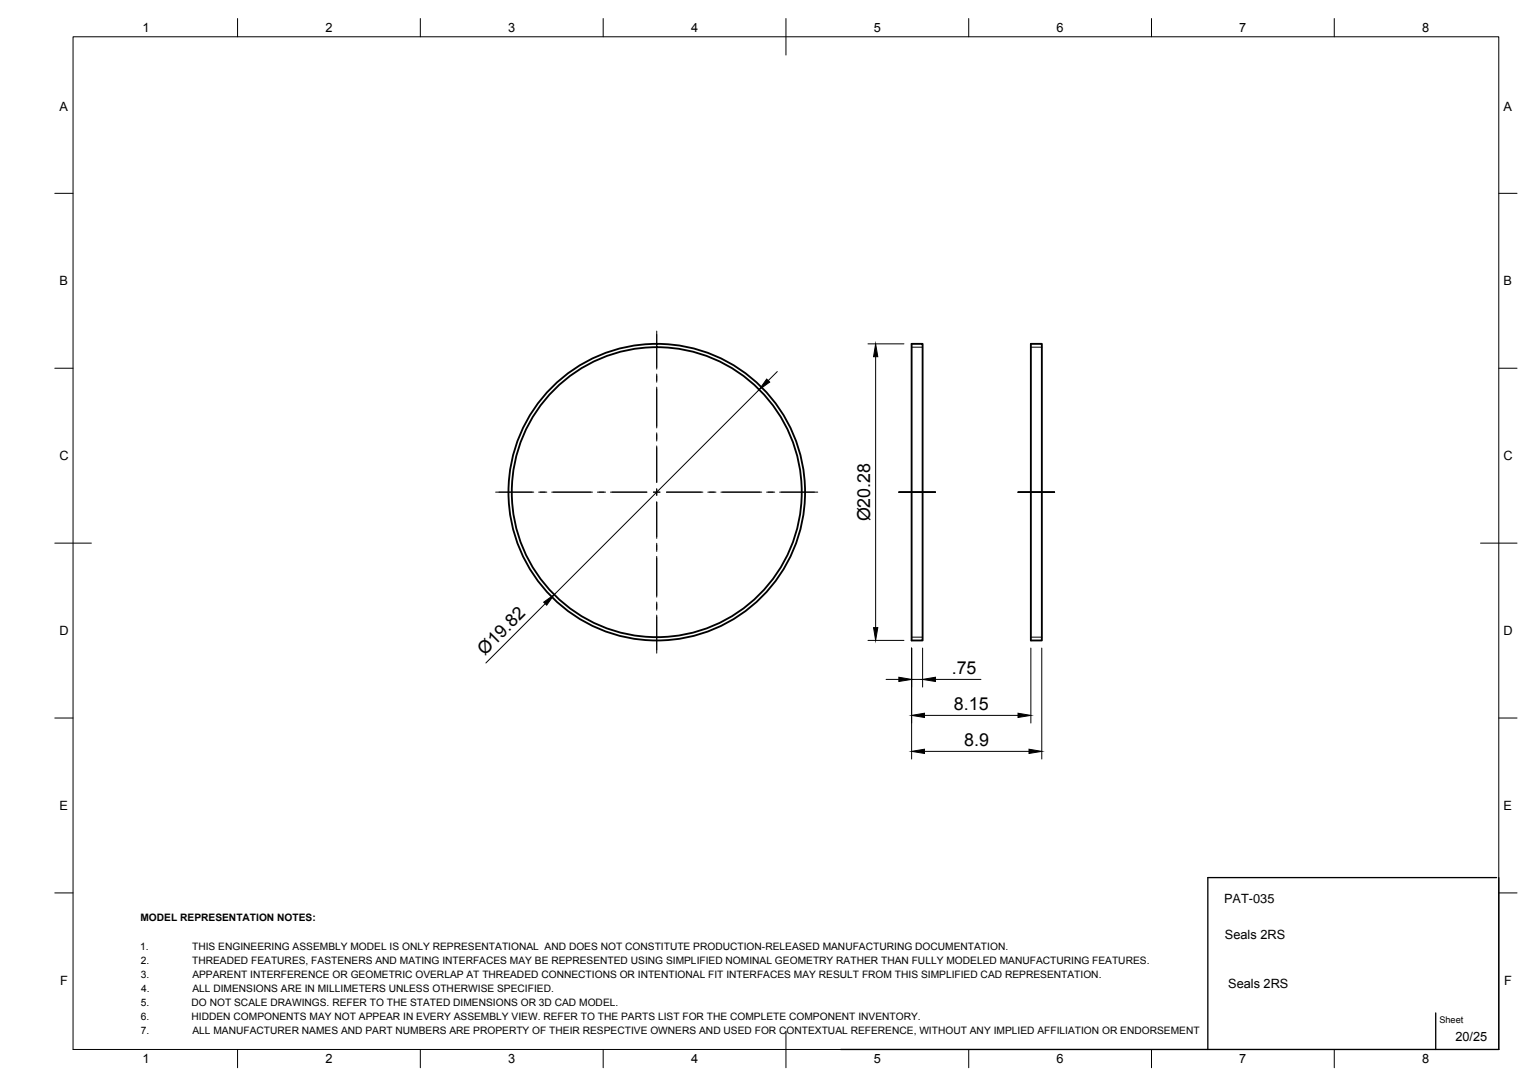
ISO-10303-21;
HEADER;
/* Generated by software containing ST-Developer
 * from STEP Tools, Inc. (www.steptools.com) 
 */

FILE_DESCRIPTION(
/* description */ ('Five-roller gravity conveyor'),
/* implementation_level */ '2;1');

FILE_NAME(
/* name */ 'Seals 2RS.step',
/* time_stamp */ '2026-10-29T15:36:43-07:00',
/* author */ (''),
/* organization */ (''),
/* preprocessor_version */ 'ST-DEVELOPER v20.2',
/* originating_system */ 'Autodesk Translation Framework v15.17.0.0',
/* authorisation */ '');

FILE_SCHEMA (('AUTOMOTIVE_DESIGN { 1 0 10303 214 3 1 1 }'));
ENDSEC;

DATA;
#10=MECHANICAL_DESIGN_GEOMETRIC_PRESENTATION_REPRESENTATION('',(#329,#330),#7806);
#286=SHAPE_REPRESENTATION_RELATIONSHIP('SRR','None',#7924,#304);
#304=ADVANCED_BREP_SHAPE_REPRESENTATION('',(#354,#355),#7797);
#329=STYLED_ITEM('',(#8091),#354);
#330=STYLED_ITEM('',(#8091),#355);
#354=MANIFOLD_SOLID_BREP('Body1',#4217);
#355=MANIFOLD_SOLID_BREP('Body2',#4218);
#387=FACE_BOUND('',#1083,.T.);
#388=FACE_BOUND('',#1086,.T.);
#389=FACE_BOUND('',#1089,.T.);
#390=FACE_BOUND('',#1092,.T.);
#536=CIRCLE('',#4732,1.013815);
#537=CIRCLE('',#4733,0.991185);
#538=CIRCLE('',#4735,1.013815);
#539=CIRCLE('',#4737,0.991185);
#540=CIRCLE('',#4740,1.013815);
#541=CIRCLE('',#4741,0.991185);
#542=CIRCLE('',#4743,1.013815);
#543=CIRCLE('',#4745,0.991185);
#625=CYLINDRICAL_SURFACE('',#4734,1.013815);
#626=CYLINDRICAL_SURFACE('',#4738,0.991185);
#627=CYLINDRICAL_SURFACE('',#4742,1.013815);
#628=CYLINDRICAL_SURFACE('',#4746,0.991185);
#825=FACE_OUTER_BOUND('',#1082,.T.);
#826=FACE_OUTER_BOUND('',#1084,.T.);
#827=FACE_OUTER_BOUND('',#1085,.T.);
#828=FACE_OUTER_BOUND('',#1087,.T.);
#829=FACE_OUTER_BOUND('',#1088,.T.);
#830=FACE_OUTER_BOUND('',#1090,.T.);
#831=FACE_OUTER_BOUND('',#1091,.T.);
#832=FACE_OUTER_BOUND('',#1093,.T.);
#1082=EDGE_LOOP('',(#3608));
#1083=EDGE_LOOP('',(#3609));
#1084=EDGE_LOOP('',(#3610,#3611,#3612,#3613));
#1085=EDGE_LOOP('',(#3614));
#1086=EDGE_LOOP('',(#3615));
#1087=EDGE_LOOP('',(#3616,#3617,#3618,#3619));
#1088=EDGE_LOOP('',(#3620));
#1089=EDGE_LOOP('',(#3621));
#1090=EDGE_LOOP('',(#3622,#3623,#3624,#3625));
#1091=EDGE_LOOP('',(#3626));
#1092=EDGE_LOOP('',(#3627));
#1093=EDGE_LOOP('',(#3628,#3629,#3630,#3631));
#1467=LINE('',#7470,#1808);
#1468=LINE('',#7475,#1809);
#1469=LINE('',#7484,#1810);
#1470=LINE('',#7489,#1811);
#1808=VECTOR('',#5821,1.013815);
#1809=VECTOR('',#5828,0.991185);
#1810=VECTOR('',#5839,1.013815);
#1811=VECTOR('',#5846,0.991185);
#2150=VERTEX_POINT('',#7463);
#2151=VERTEX_POINT('',#7465);
#2152=VERTEX_POINT('',#7468);
#2153=VERTEX_POINT('',#7472);
#2154=VERTEX_POINT('',#7477);
#2155=VERTEX_POINT('',#7479);
#2156=VERTEX_POINT('',#7482);
#2157=VERTEX_POINT('',#7486);
#2647=EDGE_CURVE('',#2150,#2150,#536,.T.);
#2648=EDGE_CURVE('',#2151,#2151,#537,.T.);
#2649=EDGE_CURVE('',#2152,#2152,#538,.T.);
#2650=EDGE_CURVE('',#2152,#2150,#1467,.T.);
#2651=EDGE_CURVE('',#2153,#2153,#539,.T.);
#2652=EDGE_CURVE('',#2153,#2151,#1468,.T.);
#2653=EDGE_CURVE('',#2154,#2154,#540,.T.);
#2654=EDGE_CURVE('',#2155,#2155,#541,.T.);
#2655=EDGE_CURVE('',#2156,#2156,#542,.T.);
#2656=EDGE_CURVE('',#2156,#2154,#1469,.T.);
#2657=EDGE_CURVE('',#2157,#2157,#543,.T.);
#2658=EDGE_CURVE('',#2157,#2155,#1470,.T.);
#3608=ORIENTED_EDGE('',*,*,#2647,.F.);
#3609=ORIENTED_EDGE('',*,*,#2648,.T.);
#3610=ORIENTED_EDGE('',*,*,#2649,.F.);
#3611=ORIENTED_EDGE('',*,*,#2650,.T.);
#3612=ORIENTED_EDGE('',*,*,#2647,.T.);
#3613=ORIENTED_EDGE('',*,*,#2650,.F.);
#3614=ORIENTED_EDGE('',*,*,#2649,.T.);
#3615=ORIENTED_EDGE('',*,*,#2651,.F.);
#3616=ORIENTED_EDGE('',*,*,#2651,.T.);
#3617=ORIENTED_EDGE('',*,*,#2652,.T.);
#3618=ORIENTED_EDGE('',*,*,#2648,.F.);
#3619=ORIENTED_EDGE('',*,*,#2652,.F.);
#3620=ORIENTED_EDGE('',*,*,#2653,.F.);
#3621=ORIENTED_EDGE('',*,*,#2654,.T.);
#3622=ORIENTED_EDGE('',*,*,#2655,.F.);
#3623=ORIENTED_EDGE('',*,*,#2656,.T.);
#3624=ORIENTED_EDGE('',*,*,#2653,.T.);
#3625=ORIENTED_EDGE('',*,*,#2656,.F.);
#3626=ORIENTED_EDGE('',*,*,#2655,.T.);
#3627=ORIENTED_EDGE('',*,*,#2657,.F.);
#3628=ORIENTED_EDGE('',*,*,#2657,.T.);
#3629=ORIENTED_EDGE('',*,*,#2658,.T.);
#3630=ORIENTED_EDGE('',*,*,#2654,.F.);
#3631=ORIENTED_EDGE('',*,*,#2658,.F.);
#3939=PLANE('',#4731);
#3940=PLANE('',#4736);
#3941=PLANE('',#4739);
#3942=PLANE('',#4744);
#4140=ADVANCED_FACE('',(#825,#387),#3939,.T.);
#4141=ADVANCED_FACE('',(#826),#625,.T.);
#4142=ADVANCED_FACE('',(#827,#388),#3940,.T.);
#4143=ADVANCED_FACE('',(#828),#626,.F.);
#4144=ADVANCED_FACE('',(#829,#389),#3941,.T.);
#4145=ADVANCED_FACE('',(#830),#627,.T.);
#4146=ADVANCED_FACE('',(#831,#390),#3942,.T.);
#4147=ADVANCED_FACE('',(#832),#628,.F.);
#4217=CLOSED_SHELL('',(#4140,#4141,#4142,#4143));
#4218=CLOSED_SHELL('',(#4144,#4145,#4146,#4147));
#4730=AXIS2_PLACEMENT_3D('',#7461,#5809,#5810);
#4731=AXIS2_PLACEMENT_3D('',#7462,#5811,#5812);
#4732=AXIS2_PLACEMENT_3D('',#7464,#5813,#5814);
#4733=AXIS2_PLACEMENT_3D('',#7466,#5815,#5816);
#4734=AXIS2_PLACEMENT_3D('',#7467,#5817,#5818);
#4735=AXIS2_PLACEMENT_3D('',#7469,#5819,#5820);
#4736=AXIS2_PLACEMENT_3D('',#7471,#5822,#5823);
#4737=AXIS2_PLACEMENT_3D('',#7473,#5824,#5825);
#4738=AXIS2_PLACEMENT_3D('',#7474,#5826,#5827);
#4739=AXIS2_PLACEMENT_3D('',#7476,#5829,#5830);
#4740=AXIS2_PLACEMENT_3D('',#7478,#5831,#5832);
#4741=AXIS2_PLACEMENT_3D('',#7480,#5833,#5834);
#4742=AXIS2_PLACEMENT_3D('',#7481,#5835,#5836);
#4743=AXIS2_PLACEMENT_3D('',#7483,#5837,#5838);
#4744=AXIS2_PLACEMENT_3D('',#7485,#5840,#5841);
#4745=AXIS2_PLACEMENT_3D('',#7487,#5842,#5843);
#4746=AXIS2_PLACEMENT_3D('',#7488,#5844,#5845);
#5809=DIRECTION('axis',(0.,0.,1.));
#5810=DIRECTION('refdir',(1.,0.,0.));
#5811=DIRECTION('center_axis',(0.,1.,0.));
#5812=DIRECTION('ref_axis',(0.,0.,1.));
#5813=DIRECTION('center_axis',(0.,-1.,0.));
#5814=DIRECTION('ref_axis',(1.,0.,0.));
#5815=DIRECTION('center_axis',(0.,-1.,0.));
#5816=DIRECTION('ref_axis',(1.,0.,0.));
#5817=DIRECTION('center_axis',(0.,-1.,0.));
#5818=DIRECTION('ref_axis',(1.,0.,0.));
#5819=DIRECTION('center_axis',(0.,-1.,0.));
#5820=DIRECTION('ref_axis',(1.,0.,0.));
#5821=DIRECTION('',(0.,1.,0.));
#5822=DIRECTION('center_axis',(0.,-1.,0.));
#5823=DIRECTION('ref_axis',(0.,0.,-1.));
#5824=DIRECTION('center_axis',(0.,-1.,0.));
#5825=DIRECTION('ref_axis',(1.,0.,0.));
#5826=DIRECTION('center_axis',(0.,-1.,0.));
#5827=DIRECTION('ref_axis',(1.,0.,0.));
#5828=DIRECTION('',(0.,1.,0.));
#5829=DIRECTION('center_axis',(0.,1.,0.));
#5830=DIRECTION('ref_axis',(0.,0.,1.));
#5831=DIRECTION('center_axis',(0.,-1.,0.));
#5832=DIRECTION('ref_axis',(1.,0.,0.));
#5833=DIRECTION('center_axis',(0.,-1.,0.));
#5834=DIRECTION('ref_axis',(1.,0.,0.));
#5835=DIRECTION('center_axis',(0.,-1.,0.));
#5836=DIRECTION('ref_axis',(1.,0.,0.));
#5837=DIRECTION('center_axis',(0.,-1.,0.));
#5838=DIRECTION('ref_axis',(1.,0.,0.));
#5839=DIRECTION('',(0.,1.,0.));
#5840=DIRECTION('center_axis',(0.,-1.,0.));
#5841=DIRECTION('ref_axis',(0.,0.,-1.));
#5842=DIRECTION('center_axis',(0.,-1.,0.));
#5843=DIRECTION('ref_axis',(1.,0.,0.));
#5844=DIRECTION('center_axis',(0.,-1.,0.));
#5845=DIRECTION('ref_axis',(1.,0.,0.));
#5846=DIRECTION('',(0.,1.,0.));
#7461=CARTESIAN_POINT('',(0.,0.,0.));
#7462=CARTESIAN_POINT('Origin',(1.013815,0.445,0.));
#7463=CARTESIAN_POINT('',(-1.013815,0.445,-1.24156529467757E-16));
#7464=CARTESIAN_POINT('Origin',(0.,0.445,0.));
#7465=CARTESIAN_POINT('',(-0.991185,0.445,-1.21385153761287E-16));
#7466=CARTESIAN_POINT('Origin',(0.,0.445,0.));
#7467=CARTESIAN_POINT('Origin',(0.,0.4075,0.));
#7468=CARTESIAN_POINT('',(-1.013815,0.37,-1.24156529467757E-16));
#7469=CARTESIAN_POINT('Origin',(0.,0.37,0.));
#7470=CARTESIAN_POINT('',(-1.013815,0.4075,-1.24156529467757E-16));
#7471=CARTESIAN_POINT('Origin',(0.991185,0.37,0.));
#7472=CARTESIAN_POINT('',(-0.991185,0.37,-1.21385153761287E-16));
#7473=CARTESIAN_POINT('Origin',(0.,0.37,0.));
#7474=CARTESIAN_POINT('Origin',(0.,0.4075,0.));
#7475=CARTESIAN_POINT('',(-0.991185,0.4075,-1.21385153761287E-16));
#7476=CARTESIAN_POINT('Origin',(1.013815,-0.37,0.));
#7477=CARTESIAN_POINT('',(-1.013815,-0.37,-1.24156529467757E-16));
#7478=CARTESIAN_POINT('Origin',(0.,-0.37,0.));
#7479=CARTESIAN_POINT('',(-0.991185,-0.37,-1.21385153761287E-16));
#7480=CARTESIAN_POINT('Origin',(0.,-0.37,0.));
#7481=CARTESIAN_POINT('Origin',(0.,-0.4075,0.));
#7482=CARTESIAN_POINT('',(-1.013815,-0.445,-1.24156529467757E-16));
#7483=CARTESIAN_POINT('Origin',(0.,-0.445,0.));
#7484=CARTESIAN_POINT('',(-1.013815,-0.4075,-1.24156529467757E-16));
#7485=CARTESIAN_POINT('Origin',(0.991185,-0.445,0.));
#7486=CARTESIAN_POINT('',(-0.991185,-0.445,-1.21385153761287E-16));
#7487=CARTESIAN_POINT('Origin',(0.,-0.445,0.));
#7488=CARTESIAN_POINT('Origin',(0.,-0.4075,0.));
#7489=CARTESIAN_POINT('',(-0.991185,-0.4075,-1.21385153761287E-16));
#7773=UNCERTAINTY_MEASURE_WITH_UNIT(LENGTH_MEASURE(0.001),#7807,
'DISTANCE_ACCURACY_VALUE',
'Maximum model space distance between geometric entities at asserted c
onnectivities');
#7782=UNCERTAINTY_MEASURE_WITH_UNIT(LENGTH_MEASURE(0.001),#7807,
'DISTANCE_ACCURACY_VALUE',
'Maximum model space distance between geometric entities at asserted c
onnectivities');
#7797=(
GEOMETRIC_REPRESENTATION_CONTEXT(3)
GLOBAL_UNCERTAINTY_ASSIGNED_CONTEXT((#7773))
GLOBAL_UNIT_ASSIGNED_CONTEXT((#7807,#7809,#7810))
REPRESENTATION_CONTEXT('','3D')
);
#7806=(
GEOMETRIC_REPRESENTATION_CONTEXT(3)
GLOBAL_UNCERTAINTY_ASSIGNED_CONTEXT((#7782))
GLOBAL_UNIT_ASSIGNED_CONTEXT((#7807,#7809,#7810))
REPRESENTATION_CONTEXT('','3D')
);
#7807=(
LENGTH_UNIT()
NAMED_UNIT(*)
SI_UNIT(.CENTI.,.METRE.)
);
#7809=(
NAMED_UNIT(*)
PLANE_ANGLE_UNIT()
SI_UNIT($,.RADIAN.)
);
#7810=(
NAMED_UNIT(*)
SI_UNIT($,.STERADIAN.)
SOLID_ANGLE_UNIT()
);
#7825=SHAPE_DEFINITION_REPRESENTATION(#7848,#7924);
#7848=PRODUCT_DEFINITION_SHAPE('',$,#7948);
#7924=SHAPE_REPRESENTATION('',(#4730),#7797);
#7933=PRODUCT_DEFINITION_CONTEXT('part definition',#8004,'design');
#7948=PRODUCT_DEFINITION('Seals 2RS','Seals 2RS',#7971,#7933);
#7971=PRODUCT_DEFINITION_FORMATION('',$,#8020);
#8004=APPLICATION_CONTEXT(
'Core Data for Automotive Mechanical Design Process');
#8005=PRODUCT_CONTEXT('part definition',#8004,'mechanical');
#8020=PRODUCT('Seals 2RS','Seals 2RS','Seals 2RS',(#8005));
#8085=COLOUR_RGB('Grey',0.48,0.52,0.57);
#8086=FILL_AREA_STYLE_COLOUR('',#8085);
#8087=FILL_AREA_STYLE('',(#8086));
#8088=SURFACE_STYLE_FILL_AREA(#8087);
#8089=SURFACE_SIDE_STYLE('',(#8088));
#8090=SURFACE_STYLE_USAGE(.BOTH.,#8089);
#8091=PRESENTATION_STYLE_ASSIGNMENT((#8090));
ENDSEC;
END-ISO-10303-21;
